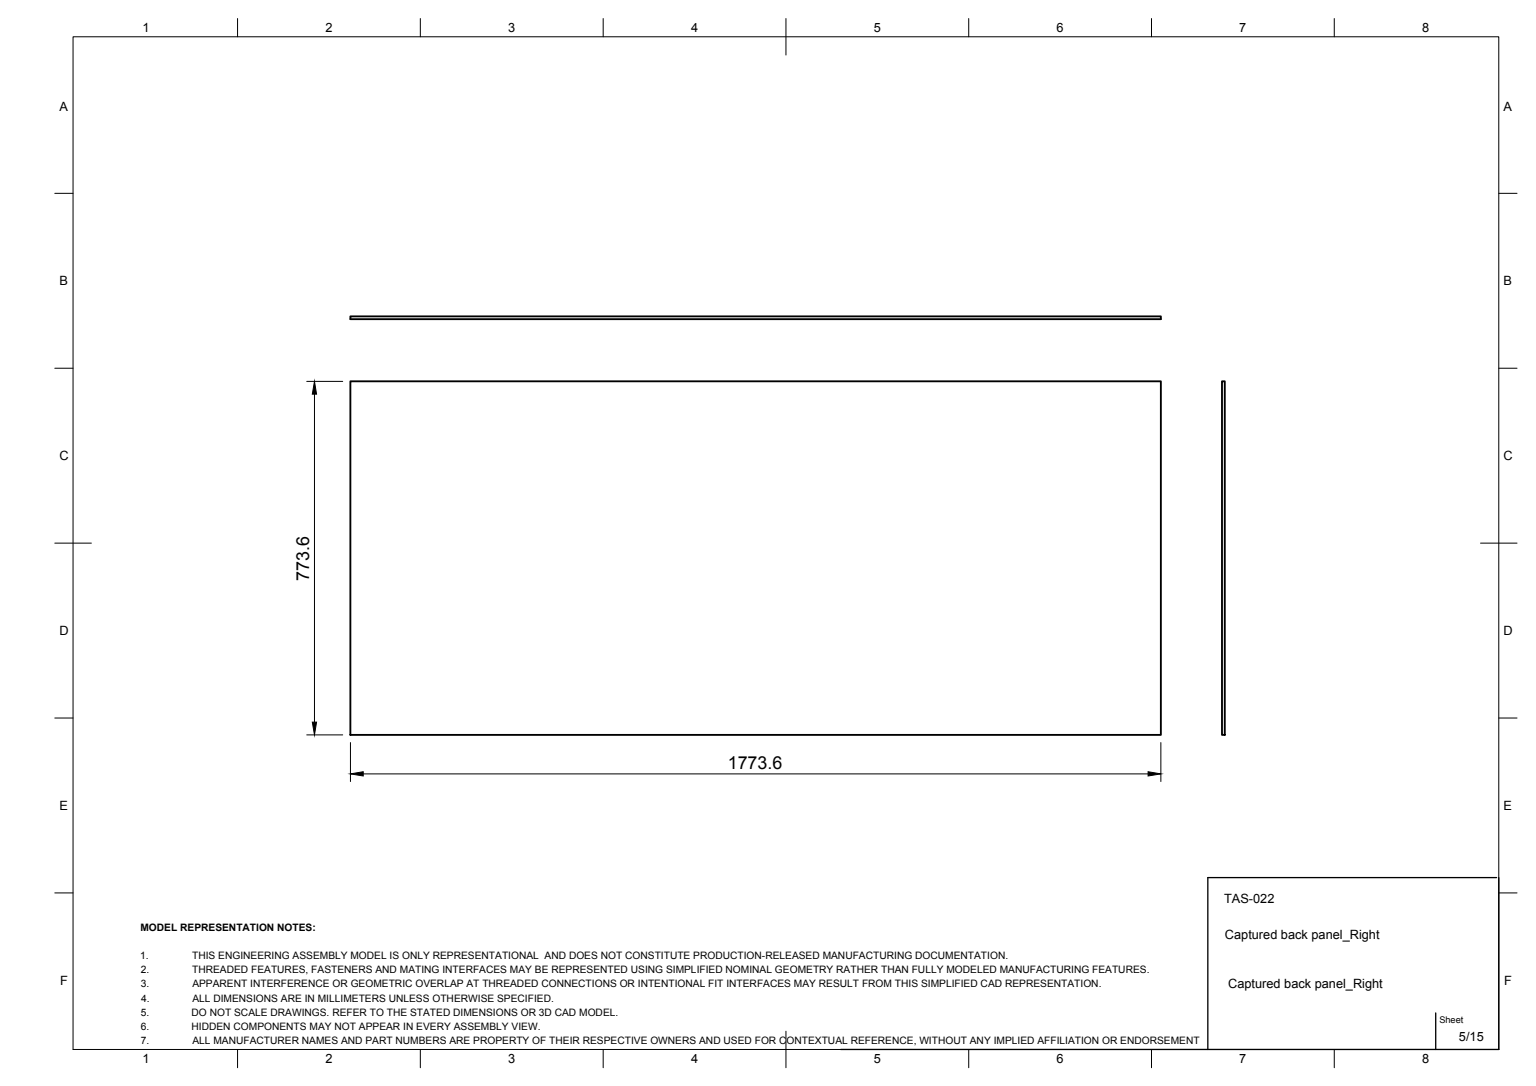
ISO-10303-21;
HEADER;
/* Generated by software containing ST-Developer
 * from STEP Tools, Inc. (www.steptools.com) 
 */

FILE_DESCRIPTION(
/* description */ (''),
/* implementation_level */ '2;1');

FILE_NAME(
/* name */ 'Captured back panel_Right.step',
/* time_stamp */ '2026-11-15T21:02:08-08:00',
/* author */ (''),
/* organization */ (''),
/* preprocessor_version */ 'ST-DEVELOPER v20.2',
/* originating_system */ 'Autodesk Translation Framework v15.17.0.0',
/* authorisation */ '');

FILE_SCHEMA (('AUTOMOTIVE_DESIGN { 1 0 10303 214 3 1 1 }'));
ENDSEC;

DATA;
#10=MECHANICAL_DESIGN_GEOMETRIC_PRESENTATION_REPRESENTATION('',(#602),#31566);
#572=SHAPE_REPRESENTATION_RELATIONSHIP('SRR','None',#31636,#587);
#587=ADVANCED_BREP_SHAPE_REPRESENTATION('',(#617),#31551);
#602=STYLED_ITEM('',(#31720),#617);
#617=MANIFOLD_SOLID_BREP('Body1',#5715);
#632=FACE_OUTER_BOUND('',#901,.T.);
#633=FACE_OUTER_BOUND('',#902,.T.);
#634=FACE_OUTER_BOUND('',#903,.T.);
#635=FACE_OUTER_BOUND('',#904,.T.);
#636=FACE_OUTER_BOUND('',#905,.T.);
#637=FACE_OUTER_BOUND('',#906,.T.);
#901=EDGE_LOOP('',(#3627,#3628,#3629,#3630));
#902=EDGE_LOOP('',(#3631,#3632,#3633,#3634));
#903=EDGE_LOOP('',(#3635,#3636,#3637,#3638));
#904=EDGE_LOOP('',(#3639,#3640,#3641,#3642));
#905=EDGE_LOOP('',(#3643,#3644,#3645,#3646));
#906=EDGE_LOOP('',(#3647,#3648,#3649,#3650));
#1206=LINE('',#7566,#1713);
#1207=LINE('',#7568,#1714);
#1208=LINE('',#7570,#1715);
#1209=LINE('',#7571,#1716);
#1210=LINE('',#7574,#1717);
#1211=LINE('',#7576,#1718);
#1212=LINE('',#7577,#1719);
#1213=LINE('',#7580,#1720);
#1214=LINE('',#7582,#1721);
#1215=LINE('',#7583,#1722);
#1216=LINE('',#7585,#1723);
#1217=LINE('',#7586,#1724);
#1713=VECTOR('',#6288,1.);
#1714=VECTOR('',#6289,1.);
#1715=VECTOR('',#6290,1.);
#1716=VECTOR('',#6291,1.);
#1717=VECTOR('',#6294,1.);
#1718=VECTOR('',#6295,1.);
#1719=VECTOR('',#6296,1.);
#1720=VECTOR('',#6299,1.);
#1721=VECTOR('',#6300,1.);
#1722=VECTOR('',#6301,1.);
#1723=VECTOR('',#6304,1.);
#1724=VECTOR('',#6305,1.);
#2220=VERTEX_POINT('',#7564);
#2221=VERTEX_POINT('',#7565);
#2222=VERTEX_POINT('',#7567);
#2223=VERTEX_POINT('',#7569);
#2224=VERTEX_POINT('',#7573);
#2225=VERTEX_POINT('',#7575);
#2226=VERTEX_POINT('',#7579);
#2227=VERTEX_POINT('',#7581);
#2809=EDGE_CURVE('',#2220,#2221,#1206,.T.);
#2810=EDGE_CURVE('',#2221,#2222,#1207,.T.);
#2811=EDGE_CURVE('',#2223,#2222,#1208,.T.);
#2812=EDGE_CURVE('',#2220,#2223,#1209,.T.);
#2813=EDGE_CURVE('',#2224,#2220,#1210,.T.);
#2814=EDGE_CURVE('',#2225,#2223,#1211,.T.);
#2815=EDGE_CURVE('',#2224,#2225,#1212,.T.);
#2816=EDGE_CURVE('',#2226,#2224,#1213,.T.);
#2817=EDGE_CURVE('',#2227,#2225,#1214,.T.);
#2818=EDGE_CURVE('',#2226,#2227,#1215,.T.);
#2819=EDGE_CURVE('',#2221,#2226,#1216,.T.);
#2820=EDGE_CURVE('',#2222,#2227,#1217,.T.);
#3627=ORIENTED_EDGE('',*,*,#2809,.T.);
#3628=ORIENTED_EDGE('',*,*,#2810,.T.);
#3629=ORIENTED_EDGE('',*,*,#2811,.F.);
#3630=ORIENTED_EDGE('',*,*,#2812,.F.);
#3631=ORIENTED_EDGE('',*,*,#2813,.T.);
#3632=ORIENTED_EDGE('',*,*,#2812,.T.);
#3633=ORIENTED_EDGE('',*,*,#2814,.F.);
#3634=ORIENTED_EDGE('',*,*,#2815,.F.);
#3635=ORIENTED_EDGE('',*,*,#2816,.T.);
#3636=ORIENTED_EDGE('',*,*,#2815,.T.);
#3637=ORIENTED_EDGE('',*,*,#2817,.F.);
#3638=ORIENTED_EDGE('',*,*,#2818,.F.);
#3639=ORIENTED_EDGE('',*,*,#2819,.T.);
#3640=ORIENTED_EDGE('',*,*,#2818,.T.);
#3641=ORIENTED_EDGE('',*,*,#2820,.F.);
#3642=ORIENTED_EDGE('',*,*,#2810,.F.);
#3643=ORIENTED_EDGE('',*,*,#2820,.T.);
#3644=ORIENTED_EDGE('',*,*,#2817,.T.);
#3645=ORIENTED_EDGE('',*,*,#2814,.T.);
#3646=ORIENTED_EDGE('',*,*,#2811,.T.);
#3647=ORIENTED_EDGE('',*,*,#2819,.F.);
#3648=ORIENTED_EDGE('',*,*,#2809,.F.);
#3649=ORIENTED_EDGE('',*,*,#2813,.F.);
#3650=ORIENTED_EDGE('',*,*,#2816,.F.);
#5263=PLANE('',#5898);
#5264=PLANE('',#5899);
#5265=PLANE('',#5900);
#5266=PLANE('',#5901);
#5267=PLANE('',#5902);
#5268=PLANE('',#5903);
#5446=ADVANCED_FACE('',(#632),#5263,.T.);
#5447=ADVANCED_FACE('',(#633),#5264,.T.);
#5448=ADVANCED_FACE('',(#634),#5265,.T.);
#5449=ADVANCED_FACE('',(#635),#5266,.T.);
#5450=ADVANCED_FACE('',(#636),#5267,.T.);
#5451=ADVANCED_FACE('',(#637),#5268,.F.);
#5715=CLOSED_SHELL('',(#5446,#5447,#5448,#5449,#5450,#5451));
#5897=AXIS2_PLACEMENT_3D('',#7562,#6284,#6285);
#5898=AXIS2_PLACEMENT_3D('',#7563,#6286,#6287);
#5899=AXIS2_PLACEMENT_3D('',#7572,#6292,#6293);
#5900=AXIS2_PLACEMENT_3D('',#7578,#6297,#6298);
#5901=AXIS2_PLACEMENT_3D('',#7584,#6302,#6303);
#5902=AXIS2_PLACEMENT_3D('',#7587,#6306,#6307);
#5903=AXIS2_PLACEMENT_3D('',#7588,#6308,#6309);
#6284=DIRECTION('axis',(0.,0.,1.));
#6285=DIRECTION('refdir',(1.,0.,0.));
#6286=DIRECTION('center_axis',(0.,1.,0.));
#6287=DIRECTION('ref_axis',(-1.,0.,0.));
#6288=DIRECTION('',(-1.,0.,0.));
#6289=DIRECTION('',(0.,0.,1.));
#6290=DIRECTION('',(-1.,0.,0.));
#6291=DIRECTION('',(0.,0.,1.));
#6292=DIRECTION('center_axis',(1.,0.,0.));
#6293=DIRECTION('ref_axis',(0.,1.,0.));
#6294=DIRECTION('',(0.,1.,0.));
#6295=DIRECTION('',(0.,1.,0.));
#6296=DIRECTION('',(0.,0.,1.));
#6297=DIRECTION('center_axis',(0.,-1.,0.));
#6298=DIRECTION('ref_axis',(1.,0.,0.));
#6299=DIRECTION('',(1.,0.,0.));
#6300=DIRECTION('',(1.,0.,0.));
#6301=DIRECTION('',(0.,0.,1.));
#6302=DIRECTION('center_axis',(-1.,0.,0.));
#6303=DIRECTION('ref_axis',(0.,-1.,0.));
#6304=DIRECTION('',(0.,-1.,0.));
#6305=DIRECTION('',(0.,-1.,0.));
#6306=DIRECTION('center_axis',(0.,0.,1.));
#6307=DIRECTION('ref_axis',(1.,0.,0.));
#6308=DIRECTION('center_axis',(0.,0.,1.));
#6309=DIRECTION('ref_axis',(1.,0.,0.));
#7562=CARTESIAN_POINT('',(0.,0.,0.));
#7563=CARTESIAN_POINT('Origin',(77.36,0.6,0.));
#7564=CARTESIAN_POINT('',(77.36,0.6,0.));
#7565=CARTESIAN_POINT('',(0.,0.6,0.));
#7566=CARTESIAN_POINT('',(77.36,0.6,0.));
#7567=CARTESIAN_POINT('',(0.,0.6,177.36));
#7568=CARTESIAN_POINT('',(0.,0.6,0.));
#7569=CARTESIAN_POINT('',(77.36,0.6,177.36));
#7570=CARTESIAN_POINT('',(77.36,0.6,177.36));
#7571=CARTESIAN_POINT('',(77.36,0.6,0.));
#7572=CARTESIAN_POINT('Origin',(77.36,0.,0.));
#7573=CARTESIAN_POINT('',(77.36,0.,0.));
#7574=CARTESIAN_POINT('',(77.36,0.,0.));
#7575=CARTESIAN_POINT('',(77.36,0.,177.36));
#7576=CARTESIAN_POINT('',(77.36,0.,177.36));
#7577=CARTESIAN_POINT('',(77.36,0.,0.));
#7578=CARTESIAN_POINT('Origin',(0.,0.,0.));
#7579=CARTESIAN_POINT('',(0.,0.,0.));
#7580=CARTESIAN_POINT('',(0.,0.,0.));
#7581=CARTESIAN_POINT('',(0.,0.,177.36));
#7582=CARTESIAN_POINT('',(0.,0.,177.36));
#7583=CARTESIAN_POINT('',(0.,0.,0.));
#7584=CARTESIAN_POINT('Origin',(0.,0.6,0.));
#7585=CARTESIAN_POINT('',(0.,0.6,0.));
#7586=CARTESIAN_POINT('',(0.,0.6,177.36));
#7587=CARTESIAN_POINT('Origin',(38.68,0.3,177.36));
#7588=CARTESIAN_POINT('Origin',(38.68,0.3,0.));
#31534=UNCERTAINTY_MEASURE_WITH_UNIT(LENGTH_MEASURE(0.001),#31567,
'DISTANCE_ACCURACY_VALUE',
'Maximum model space distance between geometric entities at asserted c
onnectivities');
#31549=UNCERTAINTY_MEASURE_WITH_UNIT(LENGTH_MEASURE(0.001),#31567,
'DISTANCE_ACCURACY_VALUE',
'Maximum model space distance between geometric entities at asserted c
onnectivities');
#31551=(
GEOMETRIC_REPRESENTATION_CONTEXT(3)
GLOBAL_UNCERTAINTY_ASSIGNED_CONTEXT((#31534))
GLOBAL_UNIT_ASSIGNED_CONTEXT((#31567,#31569,#31570))
REPRESENTATION_CONTEXT('','3D')
);
#31566=(
GEOMETRIC_REPRESENTATION_CONTEXT(3)
GLOBAL_UNCERTAINTY_ASSIGNED_CONTEXT((#31549))
GLOBAL_UNIT_ASSIGNED_CONTEXT((#31567,#31569,#31570))
REPRESENTATION_CONTEXT('','3D')
);
#31567=(
LENGTH_UNIT()
NAMED_UNIT(*)
SI_UNIT(.CENTI.,.METRE.)
);
#31569=(
NAMED_UNIT(*)
PLANE_ANGLE_UNIT()
SI_UNIT($,.RADIAN.)
);
#31570=(
NAMED_UNIT(*)
SI_UNIT($,.STERADIAN.)
SOLID_ANGLE_UNIT()
);
#31572=SHAPE_DEFINITION_REPRESENTATION(#31588,#31636);
#31588=PRODUCT_DEFINITION_SHAPE('',$,#31653);
#31636=SHAPE_REPRESENTATION('',(#5897),#31551);
#31651=PRODUCT_DEFINITION_CONTEXT('part definition',#31701,'design');
#31653=PRODUCT_DEFINITION('Captured back panel_Right',
'Captured back panel_Right',#31669,#31651);
#31669=PRODUCT_DEFINITION_FORMATION('',$,#31704);
#31701=APPLICATION_CONTEXT(
'Core Data for Automotive Mechanical Design Process');
#31702=PRODUCT_CONTEXT('part definition',#31701,'mechanical');
#31704=PRODUCT('Captured back panel_Right','Captured back panel_Right',
$,(#31702));
#31720=PRESENTATION_STYLE_ASSIGNMENT((#31727));
#31727=SURFACE_STYLE_USAGE(.BOTH.,#31734);
#31734=SURFACE_SIDE_STYLE('',(#31741));
#31741=SURFACE_STYLE_FILL_AREA(#31748);
#31748=FILL_AREA_STYLE('Opaque(155,165,179)',(#31755));
#31755=FILL_AREA_STYLE_COLOUR('Opaque(155,165,179)',#31762);
#31762=COLOUR_RGB('Opaque(155,165,179)',0.607843137254902,0.647058823529412,
0.701960784313725);
ENDSEC;
END-ISO-10303-21;
